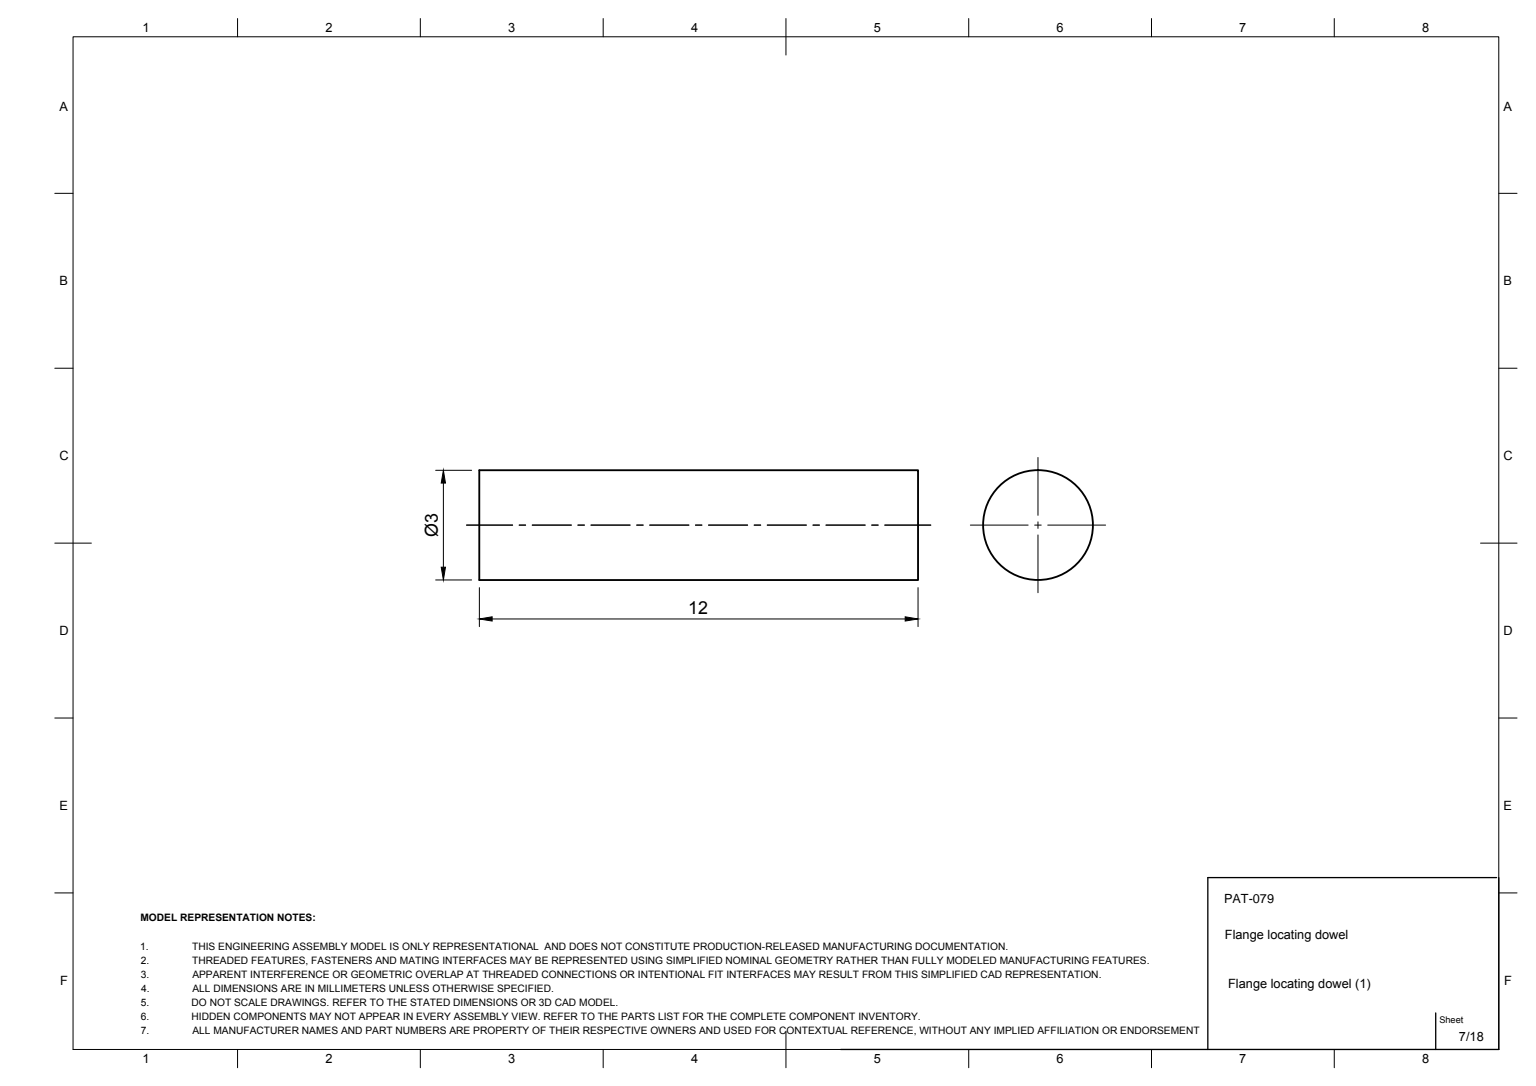
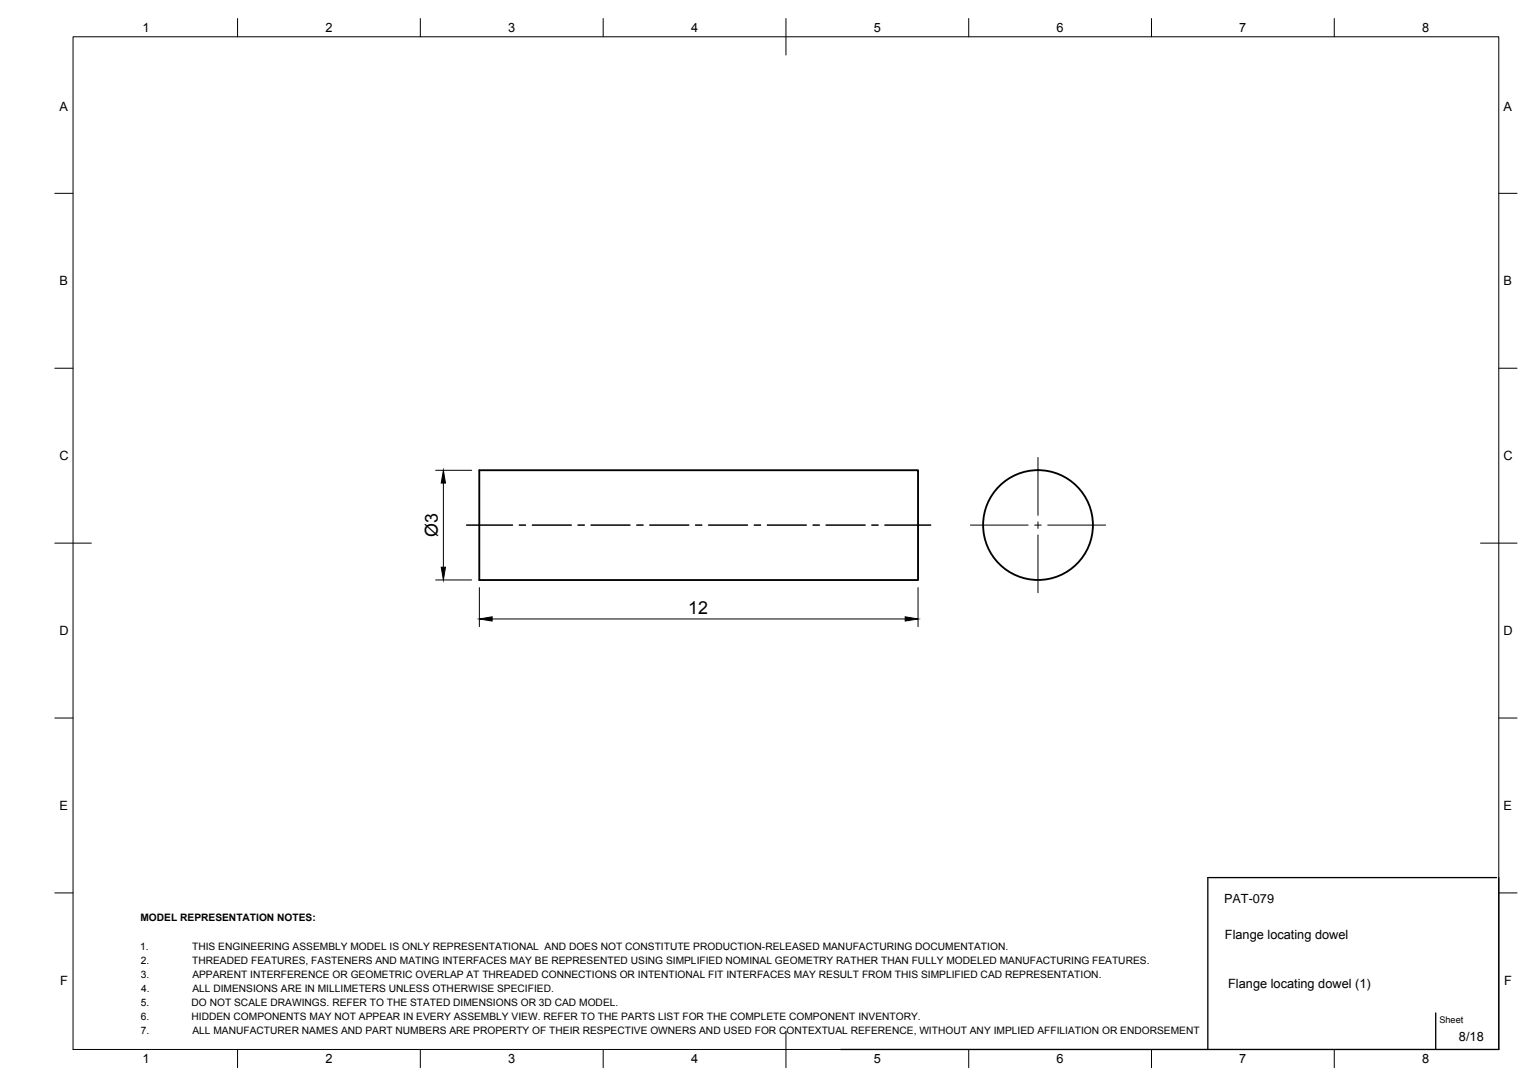
ISO-10303-21;
HEADER;
/* Generated by software containing ST-Developer
 * from STEP Tools, Inc. (www.steptools.com) 
 */

FILE_DESCRIPTION(
/* description */ ('Pipe clamp stand with threaded column'),
/* implementation_level */ '2;1');

FILE_NAME(
/* name */ 'Flange locating dowel (1).step',
/* time_stamp */ '2026-10-27T10:55:48-07:00',
/* author */ (''),
/* organization */ (''),
/* preprocessor_version */ 'ST-DEVELOPER v20.2',
/* originating_system */ 'Autodesk Translation Framework v15.17.0.0',
/* authorisation */ '');

FILE_SCHEMA (('AUTOMOTIVE_DESIGN { 1 0 10303 214 3 1 1 }'));
ENDSEC;

DATA;
#10=MECHANICAL_DESIGN_GEOMETRIC_PRESENTATION_REPRESENTATION('',(#744),#34433);
#700=SHAPE_REPRESENTATION_RELATIONSHIP('SRR','None',#34542,#722);
#722=ADVANCED_BREP_SHAPE_REPRESENTATION('',(#774),#34410);
#744=STYLED_ITEM('',(#34729),#774);
#774=MANIFOLD_SOLID_BREP('Body1',#8771);
#870=PLANE('',#9301);
#871=PLANE('',#9302);
#1263=FACE_OUTER_BOUND('',#1773,.T.);
#1264=FACE_OUTER_BOUND('',#1774,.T.);
#1265=FACE_OUTER_BOUND('',#1775,.T.);
#1773=EDGE_LOOP('',(#6773,#6774,#6775,#6776));
#1774=EDGE_LOOP('',(#6777));
#1775=EDGE_LOOP('',(#6778));
#2290=LINE('',#28028,#2907);
#2907=VECTOR('',#10453,0.15);
#3342=CIRCLE('',#9299,0.15);
#3343=CIRCLE('',#9300,0.15);
#3864=VERTEX_POINT('',#28025);
#3865=VERTEX_POINT('',#28027);
#4900=EDGE_CURVE('',#3864,#3864,#3342,.T.);
#4901=EDGE_CURVE('',#3864,#3865,#2290,.T.);
#4902=EDGE_CURVE('',#3865,#3865,#3343,.T.);
#6773=ORIENTED_EDGE('',*,*,#4900,.F.);
#6774=ORIENTED_EDGE('',*,*,#4901,.T.);
#6775=ORIENTED_EDGE('',*,*,#4902,.T.);
#6776=ORIENTED_EDGE('',*,*,#4901,.F.);
#6777=ORIENTED_EDGE('',*,*,#4900,.T.);
#6778=ORIENTED_EDGE('',*,*,#4902,.F.);
#8203=CYLINDRICAL_SURFACE('',#9298,0.15);
#8500=ADVANCED_FACE('',(#1263),#8203,.T.);
#8501=ADVANCED_FACE('',(#1264),#870,.T.);
#8502=ADVANCED_FACE('',(#1265),#871,.F.);
#8771=CLOSED_SHELL('',(#8500,#8501,#8502));
#9297=AXIS2_PLACEMENT_3D('',#28023,#10447,#10448);
#9298=AXIS2_PLACEMENT_3D('',#28024,#10449,#10450);
#9299=AXIS2_PLACEMENT_3D('',#28026,#10451,#10452);
#9300=AXIS2_PLACEMENT_3D('',#28029,#10454,#10455);
#9301=AXIS2_PLACEMENT_3D('',#28030,#10456,#10457);
#9302=AXIS2_PLACEMENT_3D('',#28031,#10458,#10459);
#10447=DIRECTION('axis',(0.,0.,1.));
#10448=DIRECTION('refdir',(1.,0.,0.));
#10449=DIRECTION('center_axis',(0.,0.,1.));
#10450=DIRECTION('ref_axis',(1.,0.,0.));
#10451=DIRECTION('center_axis',(0.,0.,1.));
#10452=DIRECTION('ref_axis',(1.,0.,0.));
#10453=DIRECTION('',(0.,0.,-1.));
#10454=DIRECTION('center_axis',(0.,0.,1.));
#10455=DIRECTION('ref_axis',(1.,0.,0.));
#10456=DIRECTION('center_axis',(0.,0.,1.));
#10457=DIRECTION('ref_axis',(1.,0.,0.));
#10458=DIRECTION('center_axis',(0.,0.,1.));
#10459=DIRECTION('ref_axis',(1.,0.,0.));
#28023=CARTESIAN_POINT('',(0.,0.,0.));
#28024=CARTESIAN_POINT('Origin',(-6.3,-1.5,0.6));
#28025=CARTESIAN_POINT('',(-6.45,-1.5,1.8));
#28026=CARTESIAN_POINT('Origin',(-6.3,-1.5,1.8));
#28027=CARTESIAN_POINT('',(-6.45,-1.5,0.6));
#28028=CARTESIAN_POINT('',(-6.45,-1.5,0.6));
#28029=CARTESIAN_POINT('Origin',(-6.3,-1.5,0.6));
#28030=CARTESIAN_POINT('Origin',(-6.3,-1.5,1.8));
#28031=CARTESIAN_POINT('Origin',(-6.3,-1.5,0.6));
#34381=UNCERTAINTY_MEASURE_WITH_UNIT(LENGTH_MEASURE(0.001),#34434,
'DISTANCE_ACCURACY_VALUE',
'Maximum model space distance between geometric entities at asserted c
onnectivities');
#34404=UNCERTAINTY_MEASURE_WITH_UNIT(LENGTH_MEASURE(0.001),#34434,
'DISTANCE_ACCURACY_VALUE',
'Maximum model space distance between geometric entities at asserted c
onnectivities');
#34410=(
GEOMETRIC_REPRESENTATION_CONTEXT(3)
GLOBAL_UNCERTAINTY_ASSIGNED_CONTEXT((#34381))
GLOBAL_UNIT_ASSIGNED_CONTEXT((#34434,#34436,#34437))
REPRESENTATION_CONTEXT('','3D')
);
#34433=(
GEOMETRIC_REPRESENTATION_CONTEXT(3)
GLOBAL_UNCERTAINTY_ASSIGNED_CONTEXT((#34404))
GLOBAL_UNIT_ASSIGNED_CONTEXT((#34434,#34436,#34437))
REPRESENTATION_CONTEXT('','3D')
);
#34434=(
LENGTH_UNIT()
NAMED_UNIT(*)
SI_UNIT(.CENTI.,.METRE.)
);
#34436=(
NAMED_UNIT(*)
PLANE_ANGLE_UNIT()
SI_UNIT($,.RADIAN.)
);
#34437=(
NAMED_UNIT(*)
SI_UNIT($,.STERADIAN.)
SOLID_ANGLE_UNIT()
);
#34443=SHAPE_DEFINITION_REPRESENTATION(#34471,#34542);
#34471=PRODUCT_DEFINITION_SHAPE('',$,#34571);
#34542=SHAPE_REPRESENTATION('',(#9297),#34410);
#34565=PRODUCT_DEFINITION_CONTEXT('part definition',#34651,'design');
#34571=PRODUCT_DEFINITION('Flange locating dowel (1)',
'Flange locating dowel (1)',#34599,#34565);
#34599=PRODUCT_DEFINITION_FORMATION('',$,#34658);
#34651=APPLICATION_CONTEXT(
'Core Data for Automotive Mechanical Design Process');
#34652=PRODUCT_CONTEXT('part definition',#34651,'mechanical');
#34658=PRODUCT('Flange locating dowel (1)','Flange locating dowel (1)',
'Flange locating dowel (1)',(#34652));
#34723=COLOUR_RGB('Light Blue',0.38,0.62,0.78);
#34724=FILL_AREA_STYLE_COLOUR('',#34723);
#34725=FILL_AREA_STYLE('',(#34724));
#34726=SURFACE_STYLE_FILL_AREA(#34725);
#34727=SURFACE_SIDE_STYLE('',(#34726));
#34728=SURFACE_STYLE_USAGE(.BOTH.,#34727);
#34729=PRESENTATION_STYLE_ASSIGNMENT((#34728));
ENDSEC;
END-ISO-10303-21;
